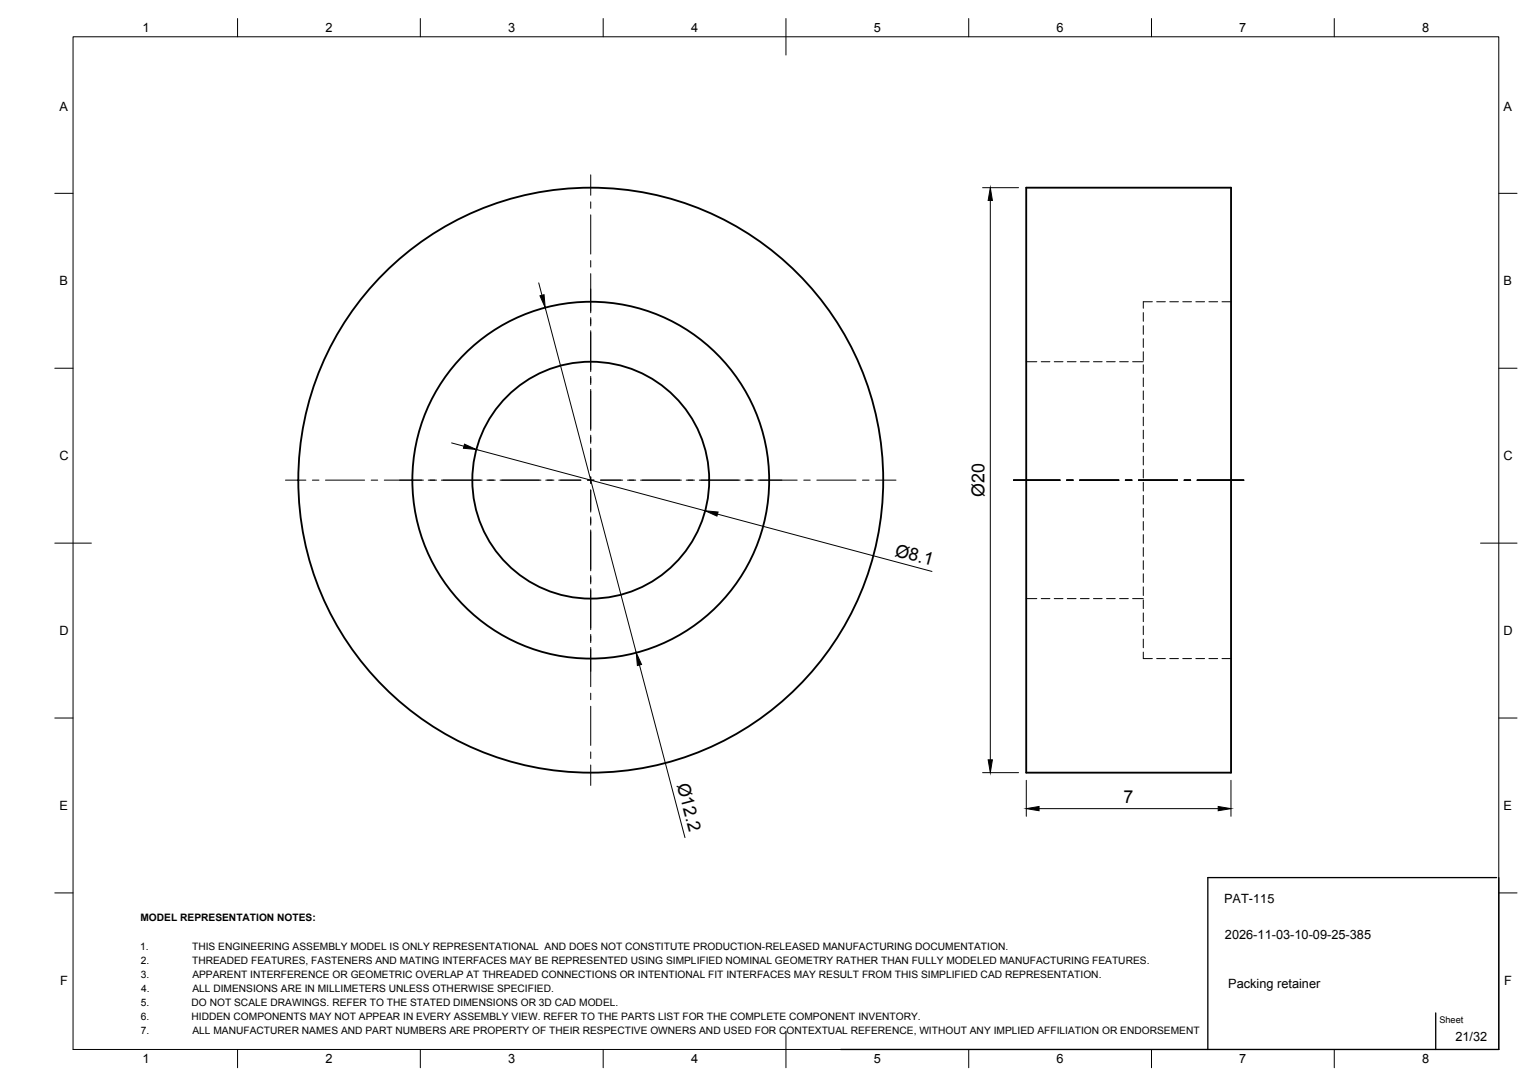
ISO-10303-21;
HEADER;
/* Generated by software containing ST-Developer
 * from STEP Tools, Inc. (www.steptools.com) 
 */

FILE_DESCRIPTION(
/* description */ ('Union bypass pipe loop'),
/* implementation_level */ '2;1');

FILE_NAME(
/* name */ 'Packing retainer.step',
/* time_stamp */ '2026-10-27T21:00:29-07:00',
/* author */ (''),
/* organization */ (''),
/* preprocessor_version */ 'ST-DEVELOPER v20.2',
/* originating_system */ 'Autodesk Translation Framework v15.17.0.0',
/* authorisation */ '');

FILE_SCHEMA (('AUTOMOTIVE_DESIGN { 1 0 10303 214 3 1 1 }'));
ENDSEC;

DATA;
#10=MECHANICAL_DESIGN_GEOMETRIC_PRESENTATION_REPRESENTATION('',(#450),#10095);
#386=SHAPE_REPRESENTATION_RELATIONSHIP('SRR','None',#10255,#418);
#418=ADVANCED_BREP_SHAPE_REPRESENTATION('',(#482),#10067);
#450=STYLED_ITEM('',(#10486),#482);
#482=MANIFOLD_SOLID_BREP('Body1',#5521);
#550=FACE_BOUND('',#1273,.T.);
#551=FACE_BOUND('',#1277,.T.);
#552=FACE_BOUND('',#1279,.T.);
#671=PLANE('',#6042);
#672=PLANE('',#6049);
#673=PLANE('',#6050);
#900=FACE_OUTER_BOUND('',#1271,.T.);
#901=FACE_OUTER_BOUND('',#1272,.T.);
#902=FACE_OUTER_BOUND('',#1274,.T.);
#903=FACE_OUTER_BOUND('',#1275,.T.);
#904=FACE_OUTER_BOUND('',#1276,.T.);
#905=FACE_OUTER_BOUND('',#1278,.T.);
#1271=EDGE_LOOP('',(#4028,#4029,#4030,#4031));
#1272=EDGE_LOOP('',(#4032));
#1273=EDGE_LOOP('',(#4033));
#1274=EDGE_LOOP('',(#4034,#4035,#4036,#4037));
#1275=EDGE_LOOP('',(#4038,#4039,#4040,#4041));
#1276=EDGE_LOOP('',(#4042));
#1277=EDGE_LOOP('',(#4043));
#1278=EDGE_LOOP('',(#4044));
#1279=EDGE_LOOP('',(#4045));
#1708=LINE('',#8743,#2084);
#1709=LINE('',#8751,#2085);
#1710=LINE('',#8756,#2086);
#2084=VECTOR('',#6976,0.61);
#2085=VECTOR('',#6987,0.405);
#2086=VECTOR('',#6992,1.);
#2435=CIRCLE('',#6040,0.61);
#2436=CIRCLE('',#6041,0.61);
#2437=CIRCLE('',#6043,0.405);
#2438=CIRCLE('',#6045,0.405);
#2439=CIRCLE('',#6047,1.);
#2440=CIRCLE('',#6048,1.);
#2727=VERTEX_POINT('',#8740);
#2728=VERTEX_POINT('',#8742);
#2729=VERTEX_POINT('',#8746);
#2730=VERTEX_POINT('',#8749);
#2731=VERTEX_POINT('',#8753);
#2732=VERTEX_POINT('',#8755);
#3212=EDGE_CURVE('',#2727,#2727,#2435,.T.);
#3213=EDGE_CURVE('',#2727,#2728,#1708,.T.);
#3214=EDGE_CURVE('',#2728,#2728,#2436,.T.);
#3215=EDGE_CURVE('',#2729,#2729,#2437,.T.);
#3216=EDGE_CURVE('',#2730,#2730,#2438,.T.);
#3217=EDGE_CURVE('',#2730,#2729,#1709,.T.);
#3218=EDGE_CURVE('',#2731,#2731,#2439,.T.);
#3219=EDGE_CURVE('',#2731,#2732,#1710,.T.);
#3220=EDGE_CURVE('',#2732,#2732,#2440,.T.);
#4028=ORIENTED_EDGE('',*,*,#3212,.F.);
#4029=ORIENTED_EDGE('',*,*,#3213,.T.);
#4030=ORIENTED_EDGE('',*,*,#3214,.T.);
#4031=ORIENTED_EDGE('',*,*,#3213,.F.);
#4032=ORIENTED_EDGE('',*,*,#3214,.F.);
#4033=ORIENTED_EDGE('',*,*,#3215,.F.);
#4034=ORIENTED_EDGE('',*,*,#3216,.F.);
#4035=ORIENTED_EDGE('',*,*,#3217,.T.);
#4036=ORIENTED_EDGE('',*,*,#3215,.T.);
#4037=ORIENTED_EDGE('',*,*,#3217,.F.);
#4038=ORIENTED_EDGE('',*,*,#3218,.F.);
#4039=ORIENTED_EDGE('',*,*,#3219,.T.);
#4040=ORIENTED_EDGE('',*,*,#3220,.T.);
#4041=ORIENTED_EDGE('',*,*,#3219,.F.);
#4042=ORIENTED_EDGE('',*,*,#3218,.T.);
#4043=ORIENTED_EDGE('',*,*,#3216,.T.);
#4044=ORIENTED_EDGE('',*,*,#3220,.F.);
#4045=ORIENTED_EDGE('',*,*,#3212,.T.);
#5106=CYLINDRICAL_SURFACE('',#6039,0.61);
#5107=CYLINDRICAL_SURFACE('',#6044,0.405);
#5108=CYLINDRICAL_SURFACE('',#6046,1.);
#5249=ADVANCED_FACE('',(#900),#5106,.F.);
#5250=ADVANCED_FACE('',(#901,#550),#671,.F.);
#5251=ADVANCED_FACE('',(#902),#5107,.F.);
#5252=ADVANCED_FACE('',(#903),#5108,.T.);
#5253=ADVANCED_FACE('',(#904,#551),#672,.T.);
#5254=ADVANCED_FACE('',(#905,#552),#673,.F.);
#5521=CLOSED_SHELL('',(#5249,#5250,#5251,#5252,#5253,#5254));
#6038=AXIS2_PLACEMENT_3D('',#8738,#6970,#6971);
#6039=AXIS2_PLACEMENT_3D('',#8739,#6972,#6973);
#6040=AXIS2_PLACEMENT_3D('',#8741,#6974,#6975);
#6041=AXIS2_PLACEMENT_3D('',#8744,#6977,#6978);
#6042=AXIS2_PLACEMENT_3D('',#8745,#6979,#6980);
#6043=AXIS2_PLACEMENT_3D('',#8747,#6981,#6982);
#6044=AXIS2_PLACEMENT_3D('',#8748,#6983,#6984);
#6045=AXIS2_PLACEMENT_3D('',#8750,#6985,#6986);
#6046=AXIS2_PLACEMENT_3D('',#8752,#6988,#6989);
#6047=AXIS2_PLACEMENT_3D('',#8754,#6990,#6991);
#6048=AXIS2_PLACEMENT_3D('',#8757,#6993,#6994);
#6049=AXIS2_PLACEMENT_3D('',#8758,#6995,#6996);
#6050=AXIS2_PLACEMENT_3D('',#8759,#6997,#6998);
#6970=DIRECTION('axis',(0.,0.,1.));
#6971=DIRECTION('refdir',(1.,0.,0.));
#6972=DIRECTION('center_axis',(0.,0.,1.));
#6973=DIRECTION('ref_axis',(1.,0.,0.));
#6974=DIRECTION('center_axis',(0.,0.,1.));
#6975=DIRECTION('ref_axis',(1.,0.,0.));
#6976=DIRECTION('',(0.,0.,1.));
#6977=DIRECTION('center_axis',(0.,0.,1.));
#6978=DIRECTION('ref_axis',(1.,0.,0.));
#6979=DIRECTION('center_axis',(0.,0.,1.));
#6980=DIRECTION('ref_axis',(1.,0.,0.));
#6981=DIRECTION('center_axis',(0.,0.,-1.));
#6982=DIRECTION('ref_axis',(1.,0.,0.));
#6983=DIRECTION('center_axis',(0.,0.,1.));
#6984=DIRECTION('ref_axis',(1.,0.,0.));
#6985=DIRECTION('center_axis',(0.,0.,-1.));
#6986=DIRECTION('ref_axis',(1.,0.,0.));
#6987=DIRECTION('',(0.,0.,-1.));
#6988=DIRECTION('center_axis',(0.,0.,1.));
#6989=DIRECTION('ref_axis',(1.,0.,0.));
#6990=DIRECTION('center_axis',(0.,0.,1.));
#6991=DIRECTION('ref_axis',(1.,0.,0.));
#6992=DIRECTION('',(0.,0.,-1.));
#6993=DIRECTION('center_axis',(0.,0.,1.));
#6994=DIRECTION('ref_axis',(1.,0.,0.));
#6995=DIRECTION('center_axis',(0.,0.,1.));
#6996=DIRECTION('ref_axis',(1.,0.,0.));
#6997=DIRECTION('center_axis',(0.,0.,1.));
#6998=DIRECTION('ref_axis',(1.,0.,0.));
#8738=CARTESIAN_POINT('',(0.,0.,0.));
#8739=CARTESIAN_POINT('Origin',(0.,0.,7.9));
#8740=CARTESIAN_POINT('',(-0.61,-7.47034547479885E-17,8.));
#8741=CARTESIAN_POINT('Origin',(0.,0.,8.));
#8742=CARTESIAN_POINT('',(-0.61,-7.47034547479885E-17,8.3));
#8743=CARTESIAN_POINT('',(-0.61,-7.47034547479885E-17,7.9));
#8744=CARTESIAN_POINT('Origin',(0.,0.,8.3));
#8745=CARTESIAN_POINT('Origin',(0.,0.,8.3));
#8746=CARTESIAN_POINT('',(-0.405,4.95981953654678E-17,8.3));
#8747=CARTESIAN_POINT('Origin',(0.,0.,8.3));
#8748=CARTESIAN_POINT('Origin',(0.,0.,8.));
#8749=CARTESIAN_POINT('',(-0.405,-4.95981953654678E-17,8.7));
#8750=CARTESIAN_POINT('Origin',(0.,0.,8.7));
#8751=CARTESIAN_POINT('',(-0.405,-4.95981953654678E-17,8.));
#8752=CARTESIAN_POINT('Origin',(0.,0.,8.));
#8753=CARTESIAN_POINT('',(-1.,-1.22464679914735E-16,8.7));
#8754=CARTESIAN_POINT('Origin',(0.,0.,8.7));
#8755=CARTESIAN_POINT('',(-1.,-1.22464679914735E-16,8.));
#8756=CARTESIAN_POINT('',(-1.,-1.22464679914735E-16,8.));
#8757=CARTESIAN_POINT('Origin',(0.,0.,8.));
#8758=CARTESIAN_POINT('Origin',(0.,0.,8.7));
#8759=CARTESIAN_POINT('Origin',(0.,0.,8.));
#10030=UNCERTAINTY_MEASURE_WITH_UNIT(LENGTH_MEASURE(0.001),#10096,
'DISTANCE_ACCURACY_VALUE',
'Maximum model space distance between geometric entities at asserted c
onnectivities');
#10058=UNCERTAINTY_MEASURE_WITH_UNIT(LENGTH_MEASURE(0.001),#10096,
'DISTANCE_ACCURACY_VALUE',
'Maximum model space distance between geometric entities at asserted c
onnectivities');
#10067=(
GEOMETRIC_REPRESENTATION_CONTEXT(3)
GLOBAL_UNCERTAINTY_ASSIGNED_CONTEXT((#10030))
GLOBAL_UNIT_ASSIGNED_CONTEXT((#10096,#10098,#10099))
REPRESENTATION_CONTEXT('','3D')
);
#10095=(
GEOMETRIC_REPRESENTATION_CONTEXT(3)
GLOBAL_UNCERTAINTY_ASSIGNED_CONTEXT((#10058))
GLOBAL_UNIT_ASSIGNED_CONTEXT((#10096,#10098,#10099))
REPRESENTATION_CONTEXT('','3D')
);
#10096=(
LENGTH_UNIT()
NAMED_UNIT(*)
SI_UNIT(.CENTI.,.METRE.)
);
#10098=(
NAMED_UNIT(*)
PLANE_ANGLE_UNIT()
SI_UNIT($,.RADIAN.)
);
#10099=(
NAMED_UNIT(*)
SI_UNIT($,.STERADIAN.)
SOLID_ANGLE_UNIT()
);
#10108=SHAPE_DEFINITION_REPRESENTATION(#10144,#10255);
#10144=PRODUCT_DEFINITION_SHAPE('',$,#10292);
#10255=SHAPE_REPRESENTATION('',(#6038),#10067);
#10283=PRODUCT_DEFINITION_CONTEXT('part definition',#10393,'design');
#10292=PRODUCT_DEFINITION('Packing retainer','Packing retainer',#10328,
#10283);
#10328=PRODUCT_DEFINITION_FORMATION('',$,#10403);
#10393=APPLICATION_CONTEXT(
'Core Data for Automotive Mechanical Design Process');
#10394=PRODUCT_CONTEXT('part definition',#10393,'mechanical');
#10403=PRODUCT('Packing retainer','Packing retainer','Packing retainer',
(#10394));
#10480=COLOUR_RGB('Light Blue',0.38,0.62,0.78);
#10481=FILL_AREA_STYLE_COLOUR('',#10480);
#10482=FILL_AREA_STYLE('',(#10481));
#10483=SURFACE_STYLE_FILL_AREA(#10482);
#10484=SURFACE_SIDE_STYLE('',(#10483));
#10485=SURFACE_STYLE_USAGE(.BOTH.,#10484);
#10486=PRESENTATION_STYLE_ASSIGNMENT((#10485));
ENDSEC;
END-ISO-10303-21;
